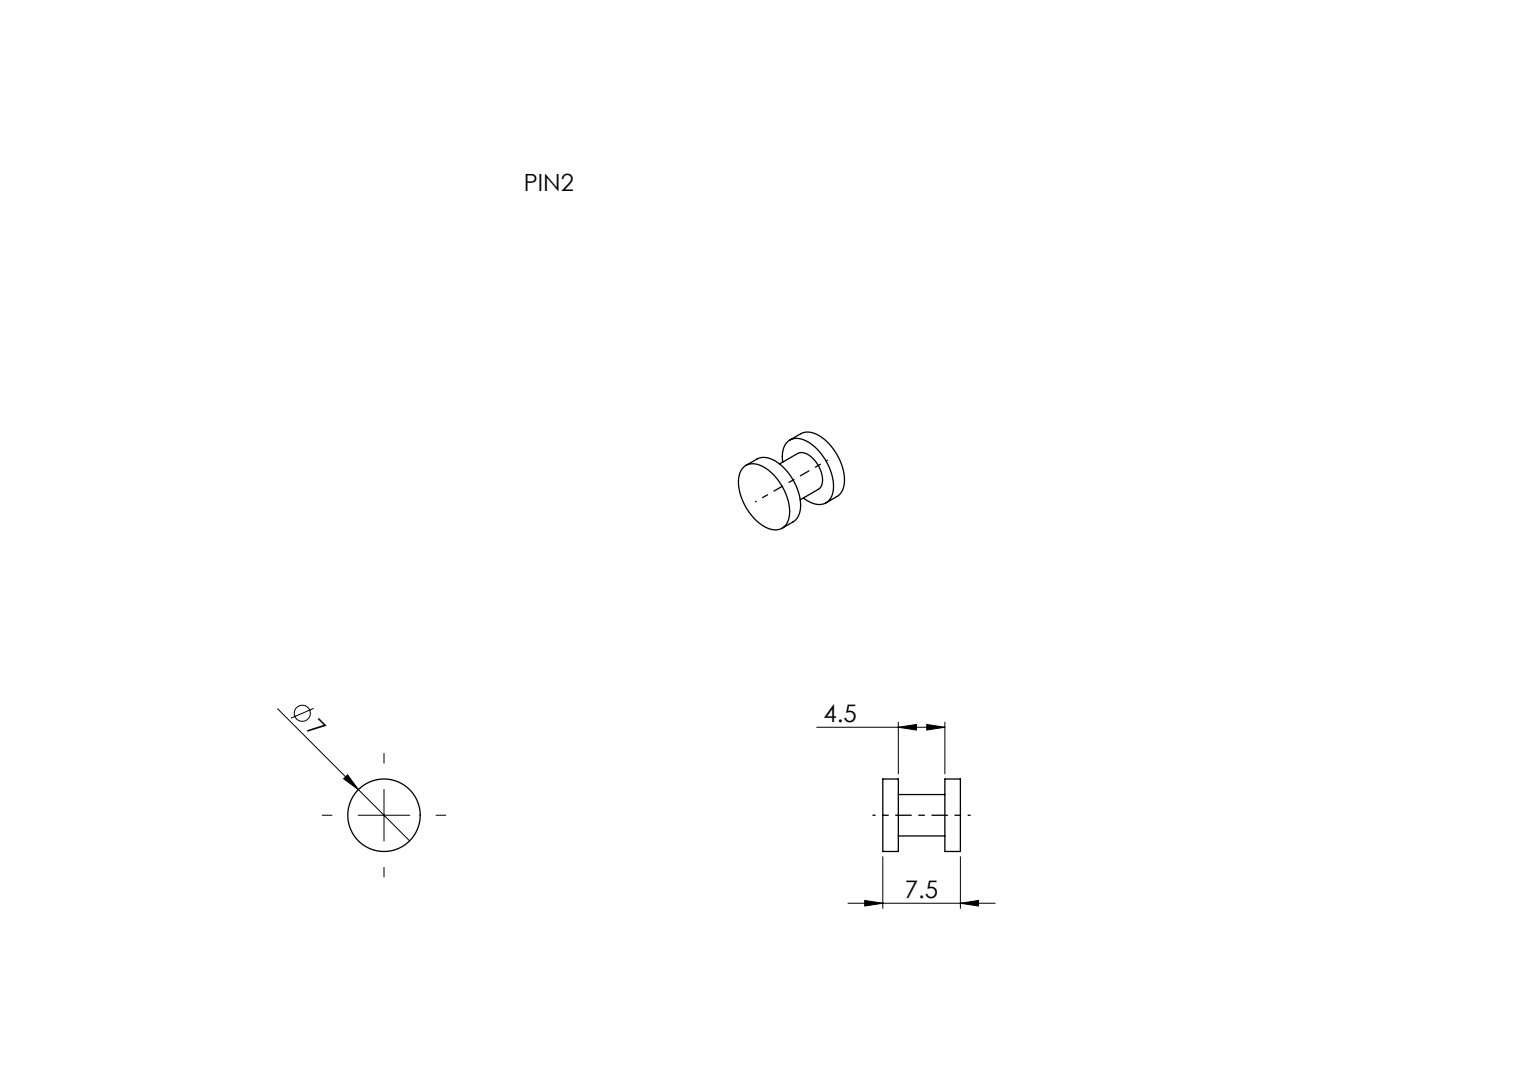
ISO-10303-21;
HEADER;
FILE_DESCRIPTION (('STEP AP214'),
    '1' );
FILE_NAME ('pin2.step',
    '2026-10-08T13:56:24',
    ( '' ),
    ( '' ),
    'SwSTEP 2.0',
    'SolidWorks 2026',
    '' );
FILE_SCHEMA (( 'AUTOMOTIVE_DESIGN' ));
ENDSEC;

DATA;
#14=CARTESIAN_POINT ( 'NONE',  ( 19.99999999999956657, -8.786575603324269439E-13, 0.000000000000000000 ) ) ;
#84=FACE_OUTER_BOUND ( 'NONE', #4287, .T. ) ;
#182=SHAPE_REPRESENTATION_RELATIONSHIP ( 'NONE' , 'NONE' ,  #1906, #2911 ) ;
#374=DIRECTION ( 'NONE',  ( 0.000000000000000000, 0.000000000000000000, 1.000000000000000000 ) ) ;
#468=FACE_BOUND ( 'NONE', #14883, .T. ) ;
#509=VERTEX_POINT ( 'NONE', #3119 ) ;
#686=SURFACE_STYLE_USAGE ( .BOTH. , #1964 ) ;
#717=VERTEX_POINT ( 'NONE', #15361 ) ;
#886=ORIENTED_EDGE ( 'NONE', *, *, #12520, .T. ) ;
#920=( NAMED_UNIT ( * ) SI_UNIT ( $, .STERADIAN. ) SOLID_ANGLE_UNIT ( ) );
#958=AXIS2_PLACEMENT_3D ( 'NONE', #7043, #8272, #6887 ) ;
#1030=CARTESIAN_POINT ( 'NONE',  ( 19.99999999999956657, -8.786575603324269439E-13, 1.500000000000000000 ) ) ;
#1045=ORIENTED_EDGE ( 'NONE', *, *, #12820, .F. ) ;
#1068=( NAMED_UNIT ( * ) PLANE_ANGLE_UNIT ( ) SI_UNIT ( $, .RADIAN. ) );
#1192=DIRECTION ( 'NONE',  ( -0.000000000000000000, -0.000000000000000000, -1.000000000000000000 ) ) ;
#1288=FACE_BOUND ( 'NONE', #3074, .T. ) ;
#1411=VERTEX_POINT ( 'NONE', #12825 ) ;
#1491=VECTOR ( 'NONE', #6393, 1000.000000000000000 ) ;
#1497=PLANE ( 'NONE',  #14932 ) ;
#1623=EDGE_CURVE ( 'NONE', #14249, #8765, #15046, .T. ) ;
#1722=UNCERTAINTY_MEASURE_WITH_UNIT (LENGTH_MEASURE( 1.000000000000000082E-05 ), #14214, 'distance_accuracy_value', 'NONE');
#1742=AXIS2_PLACEMENT_3D ( 'NONE', #3072, #7933, #4514 ) ;
#1747=CIRCLE ( 'NONE', #3542, 1.999999999999998224 ) ;
#1778=ADVANCED_FACE ( 'NONE', ( #468, #3927 ), #8956, .F. ) ;
#1855=AXIS2_PLACEMENT_3D ( 'NONE', #12682, #10206, #10293 ) ;
#1861=FACE_OUTER_BOUND ( 'NONE', #5695, .T. ) ;
#1906=SHAPE_REPRESENTATION ( 'pin2', ( #3223 ), #5534 ) ;
#1908=EDGE_LOOP ( 'NONE', ( #2842, #14498, #3720, #9541 ) ) ;
#1923=FACE_OUTER_BOUND ( 'NONE', #1908, .T. ) ;
#1964=SURFACE_SIDE_STYLE ('',( #13024 ) ) ;
#2025=AXIS2_PLACEMENT_3D ( 'NONE', #2781, #6510, #13683 ) ;
#2051=DIRECTION ( 'NONE',  ( -1.000000000000000000, 0.000000000000000000, 0.000000000000000000 ) ) ;
#2130=ADVANCED_FACE ( 'NONE', ( #1861 ), #11638, .T. ) ;
#2145=ORIENTED_EDGE ( 'NONE', *, *, #10019, .T. ) ;
#2191=VECTOR ( 'NONE', #9728, 1000.000000000000000 ) ;
#2210=CARTESIAN_POINT ( 'NONE',  ( 21.99999999999956657, -8.786575603324269439E-13, -4.500000000000000000 ) ) ;
#2404=CYLINDRICAL_SURFACE ( 'NONE', #6157, 3.499999999999999556 ) ;
#2472=ORIENTED_EDGE ( 'NONE', *, *, #5941, .F. ) ;
#2482=VECTOR ( 'NONE', #4565, 1000.000000000000000 ) ;
#2583=SURFACE_SIDE_STYLE ('',( #8003 ) ) ;
#2697=ORIENTED_EDGE ( 'NONE', *, *, #6546, .F. ) ;
#2746=FILL_AREA_STYLE_COLOUR ( '', #6315 ) ;
#2781=CARTESIAN_POINT ( 'NONE',  ( 19.99999999999956657, -8.786575603324269439E-13, -4.500000000000000000 ) ) ;
#2842=ORIENTED_EDGE ( 'NONE', *, *, #8040, .F. ) ;
#2911=ADVANCED_BREP_SHAPE_REPRESENTATION ( '', ( #3697, #3223 ), #5534 ) ;
#3017=CARTESIAN_POINT ( 'NONE',  ( 19.99999999999956657, -8.786575603324269439E-13, 1.500000000000000000 ) ) ;
#3068=AXIS2_PLACEMENT_3D ( 'NONE', #6714, #11615, #8163 ) ;
#3072=CARTESIAN_POINT ( 'NONE',  ( 19.99999999999956657, -8.786575603324269439E-13, -4.500000000000000000 ) ) ;
#3074=EDGE_LOOP ( 'NONE', ( #6900, #3628 ) ) ;
#3119=CARTESIAN_POINT ( 'NONE',  ( 17.99999999999957012, -8.784126309725975241E-13, -4.500000000000000000 ) ) ;
#3221=DIRECTION ( 'NONE',  ( 1.000000000000000000, 0.000000000000000000, 0.000000000000000000 ) ) ;
#3223=AXIS2_PLACEMENT_3D ( 'NONE', #11897, #11972, #4638 ) ;
#3329=DIRECTION ( 'NONE',  ( 0.000000000000000000, 0.000000000000000000, 1.000000000000000000 ) ) ;
#3535=ORIENTED_EDGE ( 'NONE', *, *, #12820, .T. ) ;
#3542=AXIS2_PLACEMENT_3D ( 'NONE', #11503, #374, #7890 ) ;
#3551=DIRECTION ( 'NONE',  ( 0.000000000000000000, 0.000000000000000000, 1.000000000000000000 ) ) ;
#3554=CIRCLE ( 'NONE', #13882, 3.499999999999999556 ) ;
#3628=ORIENTED_EDGE ( 'NONE', *, *, #12871, .T. ) ;
#3697=MANIFOLD_SOLID_BREP ( 'Boss-Extrude3', #13843 ) ;
#3720=ORIENTED_EDGE ( 'NONE', *, *, #13971, .T. ) ;
#3879=CARTESIAN_POINT ( 'NONE',  ( 16.49999999999956657, -8.782289339527253835E-13, -6.000000000000000000 ) ) ;
#3920=VERTEX_POINT ( 'NONE', #14896 ) ;
#3927=FACE_OUTER_BOUND ( 'NONE', #8623, .T. ) ;
#4001=APPLICATION_CONTEXT ( 'automotive_design' ) ;
#4153=ORIENTED_EDGE ( 'NONE', *, *, #15197, .T. ) ;
#4227=FACE_OUTER_BOUND ( 'NONE', #10200, .T. ) ;
#4235=DIRECTION ( 'NONE',  ( 0.000000000000000000, 0.000000000000000000, -1.000000000000000000 ) ) ;
#4287=EDGE_LOOP ( 'NONE', ( #2697, #4153, #3535, #4754 ) ) ;
#4428=( NAMED_UNIT ( * ) PLANE_ANGLE_UNIT ( ) SI_UNIT ( $, .RADIAN. ) );
#4461=EDGE_CURVE ( 'NONE', #8490, #12673, #12283, .T. ) ;
#4482=FACE_OUTER_BOUND ( 'NONE', #14641, .T. ) ;
#4514=DIRECTION ( 'NONE',  ( 1.000000000000000000, 0.000000000000000000, 0.000000000000000000 ) ) ;
#4565=DIRECTION ( 'NONE',  ( -0.000000000000000000, -0.000000000000000000, 1.000000000000000000 ) ) ;
#4638=DIRECTION ( 'NONE',  ( 1.000000000000000000, 0.000000000000000000, 0.000000000000000000 ) ) ;
#4660=ORIENTED_EDGE ( 'NONE', *, *, #9790, .T. ) ;
#4665=FACE_OUTER_BOUND ( 'NONE', #13563, .T. ) ;
#4702=( GEOMETRIC_REPRESENTATION_CONTEXT ( 3 ) GLOBAL_UNCERTAINTY_ASSIGNED_CONTEXT ( ( #11448 ) ) GLOBAL_UNIT_ASSIGNED_CONTEXT ( ( #14334, #1068, #920 ) ) REPRESENTATION_CONTEXT ( 'NONE', 'WORKASPACE' ) );
#4754=ORIENTED_EDGE ( 'NONE', *, *, #15220, .F. ) ;
#4828=DIRECTION ( 'NONE',  ( 0.000000000000000000, 0.000000000000000000, 1.000000000000000000 ) ) ;
#4922=STYLED_ITEM ( 'NONE', ( #6909 ), #3697 ) ;
#4974=ORIENTED_EDGE ( 'NONE', *, *, #4999, .F. ) ;
#4999=EDGE_CURVE ( 'NONE', #14811, #10919, #14396, .T. ) ;
#5002=DIRECTION ( 'NONE',  ( -0.000000000000000000, -0.000000000000000000, -1.000000000000000000 ) ) ;
#5049=FACE_OUTER_BOUND ( 'NONE', #14235, .T. ) ;
#5110=SHAPE_DEFINITION_REPRESENTATION ( #12976, #1906 ) ;
#5172=DIRECTION ( 'NONE',  ( 0.000000000000000000, 0.000000000000000000, 1.000000000000000000 ) ) ;
#5243=ADVANCED_FACE ( 'NONE', ( #4227 ), #9170, .T. ) ;
#5350=CARTESIAN_POINT ( 'NONE',  ( 23.49999999999956657, -8.782289339527253835E-13, 0.000000000000000000 ) ) ;
#5393=DIRECTION ( 'NONE',  ( -1.000000000000000000, 0.000000000000000000, -0.000000000000000000 ) ) ;
#5534=( GEOMETRIC_REPRESENTATION_CONTEXT ( 3 ) GLOBAL_UNCERTAINTY_ASSIGNED_CONTEXT ( ( #13845 ) ) GLOBAL_UNIT_ASSIGNED_CONTEXT ( ( #10499, #4428, #5644 ) ) REPRESENTATION_CONTEXT ( 'NONE', 'WORKASPACE' ) );
#5562=( NAMED_UNIT ( * ) SI_UNIT ( $, .STERADIAN. ) SOLID_ANGLE_UNIT ( ) );
#5644=( NAMED_UNIT ( * ) SI_UNIT ( $, .STERADIAN. ) SOLID_ANGLE_UNIT ( ) );
#5657=DIRECTION ( 'NONE',  ( 0.000000000000000000, 0.000000000000000000, 1.000000000000000000 ) ) ;
#5695=EDGE_LOOP ( 'NONE', ( #11492, #9511 ) ) ;
#5769=CARTESIAN_POINT ( 'NONE',  ( 19.99999999999956657, -8.786575603324269439E-13, -6.000000000000000000 ) ) ;
#5834=CARTESIAN_POINT ( 'NONE',  ( 16.49999999999956657, -8.782289339527253835E-13, -6.000000000000000000 ) ) ;
#5853=DIRECTION ( 'NONE',  ( -0.000000000000000000, -0.000000000000000000, 1.000000000000000000 ) ) ;
#5941=EDGE_CURVE ( 'NONE', #6708, #3920, #1747, .T. ) ;
#6049=ORIENTED_EDGE ( 'NONE', *, *, #1623, .T. ) ;
#6088=AXIS2_PLACEMENT_3D ( 'NONE', #14470, #15536, #15372 ) ;
#6122=EDGE_CURVE ( 'NONE', #11587, #717, #10282, .T. ) ;
#6141=CARTESIAN_POINT ( 'NONE',  ( 16.49999999999956657, -8.782289339527253835E-13, -4.500000000000000000 ) ) ;
#6157=AXIS2_PLACEMENT_3D ( 'NONE', #10834, #5002, #13551 ) ;
#6172=PRODUCT_CONTEXT ( 'NONE', #4001, 'mechanical' ) ;
#6187=AXIS2_PLACEMENT_3D ( 'NONE', #5769, #5853, #8218 ) ;
#6189=DIRECTION ( 'NONE',  ( -1.000000000000000000, 0.000000000000000000, 0.000000000000000000 ) ) ;
#6233=FACE_OUTER_BOUND ( 'NONE', #11019, .T. ) ;
#6238=CARTESIAN_POINT ( 'NONE',  ( 23.49999999999956657, -8.786575603324269439E-13, -6.000000000000000000 ) ) ;
#6287=DIRECTION ( 'NONE',  ( 0.000000000000000000, 0.000000000000000000, 1.000000000000000000 ) ) ;
#6315=COLOUR_RGB ( '', 0.66274510, 0.83137255, 0.94901961) ;
#6350=CARTESIAN_POINT ( 'NONE',  ( 19.99999999999956657, -8.786575603324269439E-13, 1.500000000000000000 ) ) ;
#6367=CARTESIAN_POINT ( 'NONE',  ( 19.99999999999956657, -8.786575603324269439E-13, 0.000000000000000000 ) ) ;
#6393=DIRECTION ( 'NONE',  ( -0.000000000000000000, -0.000000000000000000, 1.000000000000000000 ) ) ;
#6506=CARTESIAN_POINT ( 'NONE',  ( 19.99999999999956657, -8.786575603324269439E-13, -6.000000000000000000 ) ) ;
#6510=DIRECTION ( 'NONE',  ( 0.000000000000000000, 0.000000000000000000, 1.000000000000000000 ) ) ;
#6522=ADVANCED_FACE ( 'NONE', ( #84 ), #2404, .T. ) ;
#6546=EDGE_CURVE ( 'NONE', #8765, #14249, #3554, .T. ) ;
#6617=AXIS2_PLACEMENT_3D ( 'NONE', #12083, #12236, #14597 ) ;
#6651=AXIS2_PLACEMENT_3D ( 'NONE', #6506, #11264, #6189 ) ;
#6708=VERTEX_POINT ( 'NONE', #15884 ) ;
#6714=CARTESIAN_POINT ( 'NONE',  ( 19.99999999999956657, -8.786575603324269439E-13, -4.500000000000000000 ) ) ;
#6872=CARTESIAN_POINT ( 'NONE',  ( 19.99999999999956657, -8.786575603324269439E-13, -4.500000000000000000 ) ) ;
#6887=DIRECTION ( 'NONE',  ( 1.000000000000000000, 0.000000000000000000, 0.000000000000000000 ) ) ;
#6900=ORIENTED_EDGE ( 'NONE', *, *, #5941, .T. ) ;
#6909=PRESENTATION_STYLE_ASSIGNMENT (( #686 ) ) ;
#6985=DIRECTION ( 'NONE',  ( -1.000000000000000000, 0.000000000000000000, 0.000000000000000000 ) ) ;
#7043=CARTESIAN_POINT ( 'NONE',  ( 19.99999999999956657, -8.786575603324269439E-13, 0.000000000000000000 ) ) ;
#7183=CYLINDRICAL_SURFACE ( 'NONE', #6617, 3.499999999999999556 ) ;
#7334=MECHANICAL_DESIGN_GEOMETRIC_PRESENTATION_REPRESENTATION('',(#14306),#13498);
#7356=CARTESIAN_POINT ( 'NONE',  ( 19.99999999999956657, -8.786575603324269439E-13, 1.500000000000000000 ) ) ;
#7432=CARTESIAN_POINT ( 'NONE',  ( 16.49999999999956657, -8.786575603324269439E-13, 1.500000000000000000 ) ) ;
#7668=DIRECTION ( 'NONE',  ( 0.000000000000000000, 0.000000000000000000, -1.000000000000000000 ) ) ;
#7682=AXIS2_PLACEMENT_3D ( 'NONE', #6367, #6287, #7824 ) ;
#7824=DIRECTION ( 'NONE',  ( 1.000000000000000000, 0.000000000000000000, 0.000000000000000000 ) ) ;
#7890=DIRECTION ( 'NONE',  ( 1.000000000000000000, 0.000000000000000000, 0.000000000000000000 ) ) ;
#7933=DIRECTION ( 'NONE',  ( 0.000000000000000000, 0.000000000000000000, 1.000000000000000000 ) ) ;
#7963=DIRECTION ( 'NONE',  ( -0.000000000000000000, -0.000000000000000000, -1.000000000000000000 ) ) ;
#8003=SURFACE_STYLE_FILL_AREA ( #15511 ) ;
#8040=EDGE_CURVE ( 'NONE', #509, #3920, #11714, .T. ) ;
#8163=DIRECTION ( 'NONE',  ( -1.000000000000000000, 0.000000000000000000, 0.000000000000000000 ) ) ;
#8200=ADVANCED_FACE ( 'NONE', ( #1288, #6233 ), #8657, .F. ) ;
#8218=DIRECTION ( 'NONE',  ( 1.000000000000000000, 0.000000000000000000, 0.000000000000000000 ) ) ;
#8224=LINE ( 'NONE', #12366, #2482 ) ;
#8272=DIRECTION ( 'NONE',  ( 0.000000000000000000, 0.000000000000000000, 1.000000000000000000 ) ) ;
#8396=EDGE_CURVE ( 'NONE', #10919, #11587, #11229, .T. ) ;
#8490=VERTEX_POINT ( 'NONE', #15596 ) ;
#8511=EDGE_CURVE ( 'NONE', #509, #1411, #8725, .T. ) ;
#8623=EDGE_LOOP ( 'NONE', ( #12715, #8912 ) ) ;
#8657=PLANE ( 'NONE',  #13592 ) ;
#8699=ADVANCED_FACE ( 'NONE', ( #1923 ), #14298, .T. ) ;
#8725=CIRCLE ( 'NONE', #1742, 1.999999999999998224 ) ;
#8765=VERTEX_POINT ( 'NONE', #9596 ) ;
#8905=PRODUCT_DEFINITION ( 'UNKNOWN', '', #13325, #11421 ) ;
#8912=ORIENTED_EDGE ( 'NONE', *, *, #6122, .F. ) ;
#8956=PLANE ( 'NONE',  #13998 ) ;
#9000=AXIS2_PLACEMENT_3D ( 'NONE', #11660, #4235, #2051 ) ;
#9170=CYLINDRICAL_SURFACE ( 'NONE', #12819, 3.499999999999999556 ) ;
#9171=ADVANCED_FACE ( 'NONE', ( #10145 ), #11183, .T. ) ;
#9251=ADVANCED_FACE ( 'NONE', ( #5049 ), #1497, .T. ) ;
#9319=CARTESIAN_POINT ( 'NONE',  ( 17.99999999999957012, -8.784126309725975241E-13, -4.500000000000000000 ) ) ;
#9357=ORIENTED_EDGE ( 'NONE', *, *, #8511, .F. ) ;
#9511=ORIENTED_EDGE ( 'NONE', *, *, #14327, .T. ) ;
#9541=ORIENTED_EDGE ( 'NONE', *, *, #12871, .F. ) ;
#9596=CARTESIAN_POINT ( 'NONE',  ( 23.49999999999956657, -8.782289339527253835E-13, 1.500000000000000000 ) ) ;
#9728=DIRECTION ( 'NONE',  ( 0.000000000000000000, 0.000000000000000000, 1.000000000000000000 ) ) ;
#9775=PRODUCT ( 'pin2', 'pin2', '', ( #6172 ) ) ;
#9790=EDGE_CURVE ( 'NONE', #1411, #509, #10817, .T. ) ;
#9880=ORIENTED_EDGE ( 'NONE', *, *, #8040, .T. ) ;
#9999=CARTESIAN_POINT ( 'NONE',  ( 19.99999999999956657, -8.786575603324269439E-13, -4.500000000000000000 ) ) ;
#10019=EDGE_CURVE ( 'NONE', #717, #11587, #11323, .T. ) ;
#10145=FACE_OUTER_BOUND ( 'NONE', #13672, .T. ) ;
#10200=EDGE_LOOP ( 'NONE', ( #14127, #10604, #11451, #10635 ) ) ;
#10206=DIRECTION ( 'NONE',  ( 0.000000000000000000, 0.000000000000000000, -1.000000000000000000 ) ) ;
#10218=ORIENTED_EDGE ( 'NONE', *, *, #14327, .F. ) ;
#10282=CIRCLE ( 'NONE', #9000, 3.499999999999999556 ) ;
#10293=DIRECTION ( 'NONE',  ( -1.000000000000000000, 0.000000000000000000, -0.000000000000000000 ) ) ;
#10430=ORIENTED_EDGE ( 'NONE', *, *, #9790, .F. ) ;
#10491=ADVANCED_FACE ( 'NONE', ( #4482 ), #10786, .T. ) ;
#10499=( LENGTH_UNIT ( ) NAMED_UNIT ( * ) SI_UNIT ( .MILLI., .METRE. ) );
#10534=ORIENTED_EDGE ( 'NONE', *, *, #13971, .F. ) ;
#10604=ORIENTED_EDGE ( 'NONE', *, *, #1623, .F. ) ;
#10635=ORIENTED_EDGE ( 'NONE', *, *, #4461, .T. ) ;
#10714=AXIS2_PLACEMENT_3D ( 'NONE', #14646, #15628, #6985 ) ;
#10766=CIRCLE ( 'NONE', #958, 3.499999999999999556 ) ;
#10770=ORIENTED_EDGE ( 'NONE', *, *, #6546, .T. ) ;
#10786=CYLINDRICAL_SURFACE ( 'NONE', #6187, 3.499999999999999556 ) ;
#10815=DIRECTION ( 'NONE',  ( 1.000000000000000000, 0.000000000000000000, 0.000000000000000000 ) ) ;
#10817=CIRCLE ( 'NONE', #14681, 1.999999999999998224 ) ;
#10834=CARTESIAN_POINT ( 'NONE',  ( 19.99999999999956657, -8.786575603324269439E-13, 1.500000000000000000 ) ) ;
#10866=MECHANICAL_DESIGN_GEOMETRIC_PRESENTATION_REPRESENTATION('',(#4922),#4702);
#10919=VERTEX_POINT ( 'NONE', #5834 ) ;
#10993=CIRCLE ( 'NONE', #6088, 1.999999999999998224 ) ;
#11019=EDGE_LOOP ( 'NONE', ( #12277, #1045 ) ) ;
#11148=DIRECTION ( 'NONE',  ( 1.000000000000000000, 0.000000000000000000, -0.000000000000000000 ) ) ;
#11183=CYLINDRICAL_SURFACE ( 'NONE', #2025, 1.999999999999998224 ) ;
#11229=LINE ( 'NONE', #3879, #1491 ) ;
#11235=( NAMED_UNIT ( * ) PLANE_ANGLE_UNIT ( ) SI_UNIT ( $, .RADIAN. ) );
#11264=DIRECTION ( 'NONE',  ( 0.000000000000000000, 0.000000000000000000, -1.000000000000000000 ) ) ;
#11269=DIRECTION ( 'NONE',  ( 0.000000000000000000, 0.000000000000000000, 1.000000000000000000 ) ) ;
#11323=CIRCLE ( 'NONE', #3068, 3.499999999999999556 ) ;
#11421=PRODUCT_DEFINITION_CONTEXT ( 'detailed design', #14873, 'design' ) ;
#11448=UNCERTAINTY_MEASURE_WITH_UNIT (LENGTH_MEASURE( 1.000000000000000082E-05 ), #14334, 'distance_accuracy_value', 'NONE');
#11451=ORIENTED_EDGE ( 'NONE', *, *, #15220, .T. ) ;
#11487=VECTOR ( 'NONE', #1192, 1000.000000000000000 ) ;
#11492=ORIENTED_EDGE ( 'NONE', *, *, #4999, .T. ) ;
#11503=CARTESIAN_POINT ( 'NONE',  ( 19.99999999999956657, -8.786575603324269439E-13, 0.000000000000000000 ) ) ;
#11587=VERTEX_POINT ( 'NONE', #6141 ) ;
#11615=DIRECTION ( 'NONE',  ( 0.000000000000000000, 0.000000000000000000, -1.000000000000000000 ) ) ;
#11638=PLANE ( 'NONE',  #1855 ) ;
#11660=CARTESIAN_POINT ( 'NONE',  ( 19.99999999999956657, -8.786575603324269439E-13, -4.500000000000000000 ) ) ;
#11714=LINE ( 'NONE', #9319, #14170 ) ;
#11731=FILL_AREA_STYLE ('',( #12946 ) ) ;
#11879=COLOUR_RGB ( '', 0.66274510, 0.83137255, 0.94901961) ;
#11897=CARTESIAN_POINT ( 'NONE',  ( 0.000000000000000000, 0.000000000000000000, 0.000000000000000000 ) ) ;
#11972=DIRECTION ( 'NONE',  ( 0.000000000000000000, 0.000000000000000000, 1.000000000000000000 ) ) ;
#12041=ORIENTED_EDGE ( 'NONE', *, *, #8396, .T. ) ;
#12083=CARTESIAN_POINT ( 'NONE',  ( 19.99999999999956657, -8.786575603324269439E-13, -6.000000000000000000 ) ) ;
#12109=ADVANCED_FACE ( 'NONE', ( #4665 ), #7183, .T. ) ;
#12182=DIRECTION ( 'NONE',  ( 0.000000000000000000, 0.000000000000000000, 1.000000000000000000 ) ) ;
#12236=DIRECTION ( 'NONE',  ( -0.000000000000000000, -0.000000000000000000, 1.000000000000000000 ) ) ;
#12263=DIRECTION ( 'NONE',  ( 1.000000000000000000, 0.000000000000000000, 0.000000000000000000 ) ) ;
#12277=ORIENTED_EDGE ( 'NONE', *, *, #4461, .F. ) ;
#12283=CIRCLE ( 'NONE', #7682, 3.499999999999999556 ) ;
#12320=AXIS2_PLACEMENT_3D ( 'NONE', #6872, #5657, #3221 ) ;
#12351=CARTESIAN_POINT ( 'NONE',  ( 19.99999999999956657, -8.786575603324269439E-13, -4.500000000000000000 ) ) ;
#12366=CARTESIAN_POINT ( 'NONE',  ( 23.49999999999956657, -8.786575603324269439E-13, -6.000000000000000000 ) ) ;
#12490=LINE ( 'NONE', #14700, #11487 ) ;
#12520=EDGE_CURVE ( 'NONE', #14811, #717, #8224, .T. ) ;
#12673=VERTEX_POINT ( 'NONE', #5350 ) ;
#12682=CARTESIAN_POINT ( 'NONE',  ( 19.99999999999956657, -8.786575603324269439E-13, -6.000000000000000000 ) ) ;
#12715=ORIENTED_EDGE ( 'NONE', *, *, #10019, .F. ) ;
#12819=AXIS2_PLACEMENT_3D ( 'NONE', #3017, #7963, #12868 ) ;
#12820=EDGE_CURVE ( 'NONE', #12673, #8490, #10766, .T. ) ;
#12825=CARTESIAN_POINT ( 'NONE',  ( 21.99999999999956657, -8.786575603324269439E-13, -4.500000000000000000 ) ) ;
#12868=DIRECTION ( 'NONE',  ( -1.000000000000000000, 0.000000000000000000, 0.000000000000000000 ) ) ;
#12871=EDGE_CURVE ( 'NONE', #3920, #6708, #10993, .T. ) ;
#12946=FILL_AREA_STYLE_COLOUR ( '', #11879 ) ;
#12976=PRODUCT_DEFINITION_SHAPE ( 'NONE', 'NONE',  #8905 ) ;
#13024=SURFACE_STYLE_FILL_AREA ( #11731 ) ;
#13267=LINE ( 'NONE', #2210, #2191 ) ;
#13281=ORIENTED_EDGE ( 'NONE', *, *, #8396, .F. ) ;
#13325=PRODUCT_DEFINITION_FORMATION_WITH_SPECIFIED_SOURCE ( 'ANY', '', #9775, .NOT_KNOWN. ) ;
#13464=AXIS2_PLACEMENT_3D ( 'NONE', #1030, #4828, #10815 ) ;
#13498=( GEOMETRIC_REPRESENTATION_CONTEXT ( 3 ) GLOBAL_UNCERTAINTY_ASSIGNED_CONTEXT ( ( #1722 ) ) GLOBAL_UNIT_ASSIGNED_CONTEXT ( ( #14214, #11235, #5562 ) ) REPRESENTATION_CONTEXT ( 'NONE', 'WORKASPACE' ) );
#13551=DIRECTION ( 'NONE',  ( -1.000000000000000000, 0.000000000000000000, 0.000000000000000000 ) ) ;
#13563=EDGE_LOOP ( 'NONE', ( #13281, #4974, #886, #2145 ) ) ;
#13592=AXIS2_PLACEMENT_3D ( 'NONE', #14, #3551, #11148 ) ;
#13641=DIRECTION ( 'NONE',  ( 1.000000000000000000, 0.000000000000000000, 0.000000000000000000 ) ) ;
#13672=EDGE_LOOP ( 'NONE', ( #4660, #9880, #2472, #10534 ) ) ;
#13683=DIRECTION ( 'NONE',  ( 1.000000000000000000, 0.000000000000000000, 0.000000000000000000 ) ) ;
#13692=ORIENTED_EDGE ( 'NONE', *, *, #6122, .T. ) ;
#13707=LINE ( 'NONE', #7432, #15633 ) ;
#13843=CLOSED_SHELL ( 'NONE', ( #10491, #6522, #9171, #8699, #5243, #9251, #8200, #12109, #2130, #1778 ) ) ;
#13845=UNCERTAINTY_MEASURE_WITH_UNIT (LENGTH_MEASURE( 1.000000000000000082E-05 ), #10499, 'distance_accuracy_value', 'NONE');
#13882=AXIS2_PLACEMENT_3D ( 'NONE', #7356, #12182, #12263 ) ;
#13971=EDGE_CURVE ( 'NONE', #1411, #6708, #13267, .T. ) ;
#13998=AXIS2_PLACEMENT_3D ( 'NONE', #9999, #7668, #5393 ) ;
#14127=ORIENTED_EDGE ( 'NONE', *, *, #15197, .F. ) ;
#14128=PRESENTATION_STYLE_ASSIGNMENT (( #15431 ) ) ;
#14170=VECTOR ( 'NONE', #3329, 1000.000000000000000 ) ;
#14214=( LENGTH_UNIT ( ) NAMED_UNIT ( * ) SI_UNIT ( .MILLI., .METRE. ) );
#14235=EDGE_LOOP ( 'NONE', ( #6049, #10770 ) ) ;
#14249=VERTEX_POINT ( 'NONE', #14484 ) ;
#14298=CYLINDRICAL_SURFACE ( 'NONE', #12320, 1.999999999999998224 ) ;
#14306=STYLED_ITEM ( 'NONE', ( #14128 ), #2911 ) ;
#14327=EDGE_CURVE ( 'NONE', #10919, #14811, #15625, .T. ) ;
#14334=( LENGTH_UNIT ( ) NAMED_UNIT ( * ) SI_UNIT ( .MILLI., .METRE. ) );
#14396=CIRCLE ( 'NONE', #6651, 3.499999999999999556 ) ;
#14470=CARTESIAN_POINT ( 'NONE',  ( 19.99999999999956657, -8.786575603324269439E-13, 0.000000000000000000 ) ) ;
#14484=CARTESIAN_POINT ( 'NONE',  ( 16.49999999999956657, -8.786575603324269439E-13, 1.500000000000000000 ) ) ;
#14498=ORIENTED_EDGE ( 'NONE', *, *, #8511, .T. ) ;
#14597=DIRECTION ( 'NONE',  ( 1.000000000000000000, 0.000000000000000000, 0.000000000000000000 ) ) ;
#14641=EDGE_LOOP ( 'NONE', ( #10218, #12041, #13692, #15327 ) ) ;
#14646=CARTESIAN_POINT ( 'NONE',  ( 19.99999999999956657, -8.786575603324269439E-13, -6.000000000000000000 ) ) ;
#14681=AXIS2_PLACEMENT_3D ( 'NONE', #12351, #5172, #13641 ) ;
#14700=CARTESIAN_POINT ( 'NONE',  ( 23.49999999999956657, -8.782289339527253835E-13, 1.500000000000000000 ) ) ;
#14811=VERTEX_POINT ( 'NONE', #6238 ) ;
#14873=APPLICATION_CONTEXT ( 'automotive_design' ) ;
#14883=EDGE_LOOP ( 'NONE', ( #10430, #9357 ) ) ;
#14896=CARTESIAN_POINT ( 'NONE',  ( 17.99999999999957012, -8.784126309725975241E-13, 0.000000000000000000 ) ) ;
#14932=AXIS2_PLACEMENT_3D ( 'NONE', #6350, #11269, #15069 ) ;
#14947=DIRECTION ( 'NONE',  ( -0.000000000000000000, -0.000000000000000000, -1.000000000000000000 ) ) ;
#15046=CIRCLE ( 'NONE', #13464, 3.499999999999999556 ) ;
#15069=DIRECTION ( 'NONE',  ( 1.000000000000000000, 0.000000000000000000, -0.000000000000000000 ) ) ;
#15197=EDGE_CURVE ( 'NONE', #8765, #12673, #12490, .T. ) ;
#15220=EDGE_CURVE ( 'NONE', #14249, #8490, #13707, .T. ) ;
#15327=ORIENTED_EDGE ( 'NONE', *, *, #12520, .F. ) ;
#15361=CARTESIAN_POINT ( 'NONE',  ( 23.49999999999956657, -8.786575603324269439E-13, -4.500000000000000000 ) ) ;
#15372=DIRECTION ( 'NONE',  ( 1.000000000000000000, 0.000000000000000000, 0.000000000000000000 ) ) ;
#15431=SURFACE_STYLE_USAGE ( .BOTH. , #2583 ) ;
#15511=FILL_AREA_STYLE ('',( #2746 ) ) ;
#15536=DIRECTION ( 'NONE',  ( 0.000000000000000000, 0.000000000000000000, 1.000000000000000000 ) ) ;
#15596=CARTESIAN_POINT ( 'NONE',  ( 16.49999999999956657, -8.786575603324269439E-13, 0.000000000000000000 ) ) ;
#15625=CIRCLE ( 'NONE', #10714, 3.499999999999999556 ) ;
#15628=DIRECTION ( 'NONE',  ( 0.000000000000000000, 0.000000000000000000, -1.000000000000000000 ) ) ;
#15633=VECTOR ( 'NONE', #14947, 1000.000000000000000 ) ;
#15884=CARTESIAN_POINT ( 'NONE',  ( 21.99999999999956657, -8.786575603324269439E-13, 0.000000000000000000 ) ) ;
ENDSEC;
END-ISO-10303-21;
